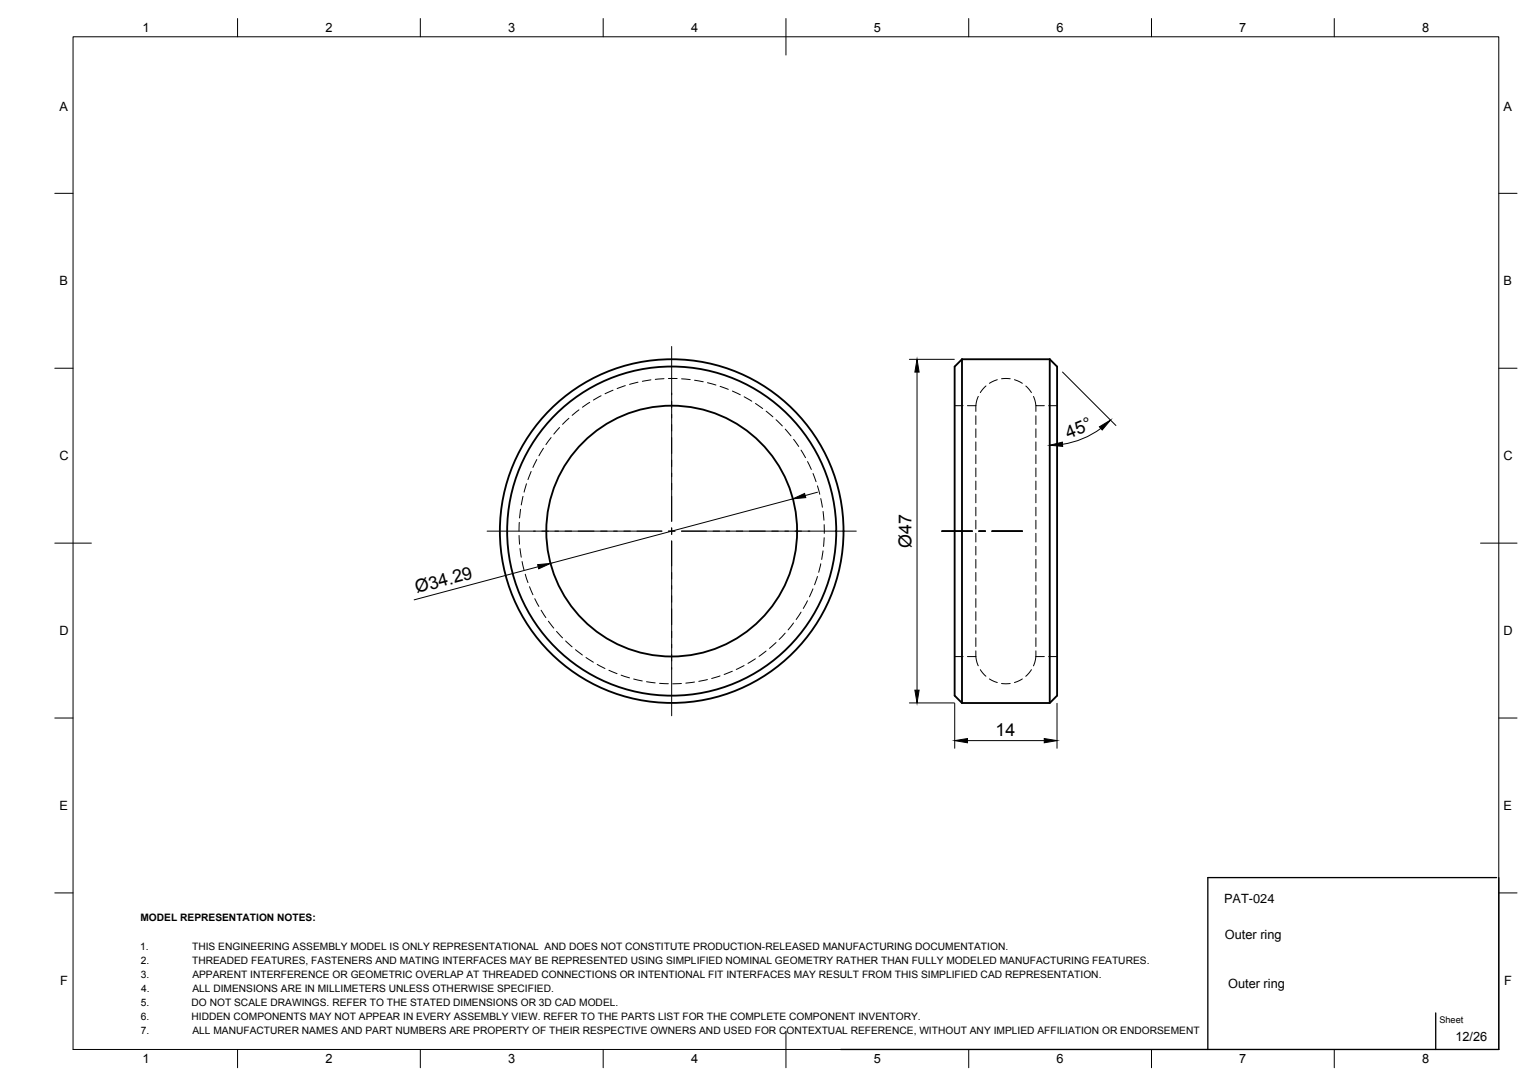
ISO-10303-21;
HEADER;
/* Generated by software containing ST-Developer
 * from STEP Tools, Inc. (www.steptools.com) 
 */

FILE_DESCRIPTION(
/* description */ ('Compact handwheel screw vise'),
/* implementation_level */ '2;1');

FILE_NAME(
/* name */ 'Outer ring.step',
/* time_stamp */ '2026-10-29T16:08:22-07:00',
/* author */ (''),
/* organization */ (''),
/* preprocessor_version */ 'ST-DEVELOPER v20.2',
/* originating_system */ 'Autodesk Translation Framework v15.17.0.0',
/* authorisation */ '');

FILE_SCHEMA (('AUTOMOTIVE_DESIGN { 1 0 10303 214 3 1 1 }'));
ENDSEC;

DATA;
#10=MECHANICAL_DESIGN_GEOMETRIC_PRESENTATION_REPRESENTATION('',(#652),#25074);
#558=TOROIDAL_SURFACE('',#8594,1.675,0.412776);
#564=CONICAL_SURFACE('',#8605,2.3,0.785398163397449);
#565=CONICAL_SURFACE('',#8609,2.3,0.785398163397449);
#596=SHAPE_REPRESENTATION_RELATIONSHIP('SRR','None',#25205,#624);
#624=ADVANCED_BREP_SHAPE_REPRESENTATION('',(#687),#25052);
#652=STYLED_ITEM('',(#25439),#687);
#687=MANIFOLD_SOLID_BREP('Body1',#8061);
#762=FACE_BOUND('',#1636,.T.);
#763=FACE_BOUND('',#1641,.T.);
#881=PLANE('',#8602);
#882=PLANE('',#8611);
#1113=FACE_OUTER_BOUND('',#1633,.T.);
#1114=FACE_OUTER_BOUND('',#1634,.T.);
#1115=FACE_OUTER_BOUND('',#1635,.T.);
#1116=FACE_OUTER_BOUND('',#1637,.T.);
#1117=FACE_OUTER_BOUND('',#1638,.T.);
#1118=FACE_OUTER_BOUND('',#1639,.T.);
#1119=FACE_OUTER_BOUND('',#1640,.T.);
#1120=FACE_OUTER_BOUND('',#1642,.T.);
#1633=EDGE_LOOP('',(#5563,#5564,#5565,#5566,#5567,#5568));
#1634=EDGE_LOOP('',(#5569,#5570,#5571,#5572,#5573));
#1635=EDGE_LOOP('',(#5574));
#1636=EDGE_LOOP('',(#5575));
#1637=EDGE_LOOP('',(#5576,#5577,#5578,#5579));
#1638=EDGE_LOOP('',(#5580,#5581,#5582,#5583));
#1639=EDGE_LOOP('',(#5584,#5585,#5586,#5587));
#1640=EDGE_LOOP('',(#5588));
#1641=EDGE_LOOP('',(#5589));
#1642=EDGE_LOOP('',(#5590,#5591,#5592,#5593,#5594));
#2184=LINE('',#11779,#2692);
#2185=LINE('',#11788,#2693);
#2186=LINE('',#11792,#2694);
#2187=LINE('',#11796,#2695);
#2188=LINE('',#11799,#2696);
#2692=VECTOR('',#9728,1.71469);
#2693=VECTOR('',#9739,2.3);
#2694=VECTOR('',#9744,2.35);
#2695=VECTOR('',#9749,2.3);
#2696=VECTOR('',#9754,1.71469);
#3158=CIRCLE('',#8595,1.71469);
#3159=CIRCLE('',#8596,1.71469);
#3160=CIRCLE('',#8597,0.412776);
#3161=CIRCLE('',#8598,1.71469);
#3162=CIRCLE('',#8599,1.71469);
#3163=CIRCLE('',#8601,1.71469);
#3164=CIRCLE('',#8603,2.25);
#3165=CIRCLE('',#8604,1.71469);
#3166=CIRCLE('',#8606,2.35);
#3167=CIRCLE('',#8608,2.35);
#3168=CIRCLE('',#8610,2.25);
#3466=VERTEX_POINT('',#11767);
#3467=VERTEX_POINT('',#11768);
#3468=VERTEX_POINT('',#11771);
#3469=VERTEX_POINT('',#11773);
#3470=VERTEX_POINT('',#11777);
#3471=VERTEX_POINT('',#11781);
#3472=VERTEX_POINT('',#11783);
#3473=VERTEX_POINT('',#11786);
#3474=VERTEX_POINT('',#11790);
#3475=VERTEX_POINT('',#11794);
#4268=EDGE_CURVE('',#3466,#3467,#3158,.T.);
#4269=EDGE_CURVE('',#3467,#3466,#3159,.T.);
#4270=EDGE_CURVE('',#3467,#3468,#3160,.T.);
#4271=EDGE_CURVE('',#3469,#3468,#3161,.T.);
#4272=EDGE_CURVE('',#3468,#3469,#3162,.T.);
#4273=EDGE_CURVE('',#3470,#3470,#3163,.T.);
#4274=EDGE_CURVE('',#3470,#3469,#2184,.T.);
#4275=EDGE_CURVE('',#3471,#3471,#3164,.T.);
#4276=EDGE_CURVE('',#3472,#3472,#3165,.T.);
#4277=EDGE_CURVE('',#3473,#3473,#3166,.T.);
#4278=EDGE_CURVE('',#3473,#3471,#2185,.T.);
#4279=EDGE_CURVE('',#3474,#3474,#3167,.T.);
#4280=EDGE_CURVE('',#3474,#3473,#2186,.T.);
#4281=EDGE_CURVE('',#3475,#3475,#3168,.T.);
#4282=EDGE_CURVE('',#3475,#3474,#2187,.T.);
#4283=EDGE_CURVE('',#3466,#3472,#2188,.T.);
#5563=ORIENTED_EDGE('',*,*,#4268,.F.);
#5564=ORIENTED_EDGE('',*,*,#4269,.F.);
#5565=ORIENTED_EDGE('',*,*,#4270,.T.);
#5566=ORIENTED_EDGE('',*,*,#4271,.F.);
#5567=ORIENTED_EDGE('',*,*,#4272,.F.);
#5568=ORIENTED_EDGE('',*,*,#4270,.F.);
#5569=ORIENTED_EDGE('',*,*,#4273,.T.);
#5570=ORIENTED_EDGE('',*,*,#4274,.T.);
#5571=ORIENTED_EDGE('',*,*,#4271,.T.);
#5572=ORIENTED_EDGE('',*,*,#4272,.T.);
#5573=ORIENTED_EDGE('',*,*,#4274,.F.);
#5574=ORIENTED_EDGE('',*,*,#4275,.F.);
#5575=ORIENTED_EDGE('',*,*,#4276,.T.);
#5576=ORIENTED_EDGE('',*,*,#4277,.F.);
#5577=ORIENTED_EDGE('',*,*,#4278,.T.);
#5578=ORIENTED_EDGE('',*,*,#4275,.T.);
#5579=ORIENTED_EDGE('',*,*,#4278,.F.);
#5580=ORIENTED_EDGE('',*,*,#4279,.F.);
#5581=ORIENTED_EDGE('',*,*,#4280,.T.);
#5582=ORIENTED_EDGE('',*,*,#4277,.T.);
#5583=ORIENTED_EDGE('',*,*,#4280,.F.);
#5584=ORIENTED_EDGE('',*,*,#4281,.F.);
#5585=ORIENTED_EDGE('',*,*,#4282,.T.);
#5586=ORIENTED_EDGE('',*,*,#4279,.T.);
#5587=ORIENTED_EDGE('',*,*,#4282,.F.);
#5588=ORIENTED_EDGE('',*,*,#4281,.T.);
#5589=ORIENTED_EDGE('',*,*,#4273,.F.);
#5590=ORIENTED_EDGE('',*,*,#4268,.T.);
#5591=ORIENTED_EDGE('',*,*,#4269,.T.);
#5592=ORIENTED_EDGE('',*,*,#4283,.T.);
#5593=ORIENTED_EDGE('',*,*,#4276,.F.);
#5594=ORIENTED_EDGE('',*,*,#4283,.F.);
#7381=CYLINDRICAL_SURFACE('',#8600,1.71469);
#7382=CYLINDRICAL_SURFACE('',#8607,2.35);
#7383=CYLINDRICAL_SURFACE('',#8612,1.71469);
#7683=ADVANCED_FACE('',(#1113),#558,.F.);
#7684=ADVANCED_FACE('',(#1114),#7381,.F.);
#7685=ADVANCED_FACE('',(#1115,#762),#881,.T.);
#7686=ADVANCED_FACE('',(#1116),#564,.T.);
#7687=ADVANCED_FACE('',(#1117),#7382,.T.);
#7688=ADVANCED_FACE('',(#1118),#565,.T.);
#7689=ADVANCED_FACE('',(#1119,#763),#882,.T.);
#7690=ADVANCED_FACE('',(#1120),#7383,.F.);
#8061=CLOSED_SHELL('',(#7683,#7684,#7685,#7686,#7687,#7688,#7689,#7690));
#8593=AXIS2_PLACEMENT_3D('',#11765,#9710,#9711);
#8594=AXIS2_PLACEMENT_3D('',#11766,#9712,#9713);
#8595=AXIS2_PLACEMENT_3D('',#11769,#9714,#9715);
#8596=AXIS2_PLACEMENT_3D('',#11770,#9716,#9717);
#8597=AXIS2_PLACEMENT_3D('',#11772,#9718,#9719);
#8598=AXIS2_PLACEMENT_3D('',#11774,#9720,#9721);
#8599=AXIS2_PLACEMENT_3D('',#11775,#9722,#9723);
#8600=AXIS2_PLACEMENT_3D('',#11776,#9724,#9725);
#8601=AXIS2_PLACEMENT_3D('',#11778,#9726,#9727);
#8602=AXIS2_PLACEMENT_3D('',#11780,#9729,#9730);
#8603=AXIS2_PLACEMENT_3D('',#11782,#9731,#9732);
#8604=AXIS2_PLACEMENT_3D('',#11784,#9733,#9734);
#8605=AXIS2_PLACEMENT_3D('',#11785,#9735,#9736);
#8606=AXIS2_PLACEMENT_3D('',#11787,#9737,#9738);
#8607=AXIS2_PLACEMENT_3D('',#11789,#9740,#9741);
#8608=AXIS2_PLACEMENT_3D('',#11791,#9742,#9743);
#8609=AXIS2_PLACEMENT_3D('',#11793,#9745,#9746);
#8610=AXIS2_PLACEMENT_3D('',#11795,#9747,#9748);
#8611=AXIS2_PLACEMENT_3D('',#11797,#9750,#9751);
#8612=AXIS2_PLACEMENT_3D('',#11798,#9752,#9753);
#9710=DIRECTION('axis',(0.,0.,1.));
#9711=DIRECTION('refdir',(1.,0.,0.));
#9712=DIRECTION('center_axis',(0.,-1.,0.));
#9713=DIRECTION('ref_axis',(0.,0.,-1.));
#9714=DIRECTION('center_axis',(0.,-1.,0.));
#9715=DIRECTION('ref_axis',(1.,0.,0.));
#9716=DIRECTION('center_axis',(0.,-1.,0.));
#9717=DIRECTION('ref_axis',(1.,0.,0.));
#9718=DIRECTION('center_axis',(1.,0.,1.22464679914735E-16));
#9719=DIRECTION('ref_axis',(-1.22464679914735E-16,0.,1.));
#9720=DIRECTION('center_axis',(0.,1.,0.));
#9721=DIRECTION('ref_axis',(1.,0.,0.));
#9722=DIRECTION('center_axis',(0.,1.,0.));
#9723=DIRECTION('ref_axis',(1.,0.,0.));
#9724=DIRECTION('center_axis',(0.,-1.,0.));
#9725=DIRECTION('ref_axis',(1.,0.,0.));
#9726=DIRECTION('center_axis',(0.,-1.,0.));
#9727=DIRECTION('ref_axis',(1.,0.,0.));
#9728=DIRECTION('',(0.,1.,0.));
#9729=DIRECTION('center_axis',(0.,1.,0.));
#9730=DIRECTION('ref_axis',(0.,0.,1.));
#9731=DIRECTION('center_axis',(0.,-1.,0.));
#9732=DIRECTION('ref_axis',(1.,0.,0.));
#9733=DIRECTION('center_axis',(0.,-1.,0.));
#9734=DIRECTION('ref_axis',(1.,0.,0.));
#9735=DIRECTION('center_axis',(0.,-1.,0.));
#9736=DIRECTION('ref_axis',(1.,0.,0.));
#9737=DIRECTION('center_axis',(0.,-1.,0.));
#9738=DIRECTION('ref_axis',(1.,0.,0.));
#9739=DIRECTION('',(0.707106781186548,0.707106781186547,8.65956056235494E-17));
#9740=DIRECTION('center_axis',(0.,-1.,0.));
#9741=DIRECTION('ref_axis',(1.,0.,0.));
#9742=DIRECTION('center_axis',(0.,-1.,0.));
#9743=DIRECTION('ref_axis',(1.,0.,0.));
#9744=DIRECTION('',(0.,1.,0.));
#9745=DIRECTION('center_axis',(0.,1.,0.));
#9746=DIRECTION('ref_axis',(1.,0.,0.));
#9747=DIRECTION('center_axis',(0.,-1.,0.));
#9748=DIRECTION('ref_axis',(1.,0.,0.));
#9749=DIRECTION('',(-0.707106781186548,0.707106781186547,-8.65956056235494E-17));
#9750=DIRECTION('center_axis',(0.,-1.,0.));
#9751=DIRECTION('ref_axis',(0.,0.,-1.));
#9752=DIRECTION('center_axis',(0.,-1.,0.));
#9753=DIRECTION('ref_axis',(1.,0.,0.));
#9754=DIRECTION('',(0.,1.,0.));
#11765=CARTESIAN_POINT('',(0.,0.,0.));
#11766=CARTESIAN_POINT('Origin',(0.,0.,0.));
#11767=CARTESIAN_POINT('',(-1.71469,0.410863395882378,-2.09988962002998E-16));
#11768=CARTESIAN_POINT('',(-2.09988962002998E-16,0.410863395882378,1.71469));
#11769=CARTESIAN_POINT('Origin',(0.,0.410863395882378,0.));
#11770=CARTESIAN_POINT('Origin',(0.,0.410863395882378,0.));
#11771=CARTESIAN_POINT('',(-2.09988962002998E-16,-0.410863395882378,1.71469));
#11772=CARTESIAN_POINT('Origin',(-2.05128338857182E-16,0.,1.675));
#11773=CARTESIAN_POINT('',(-1.71469,-0.410863395882378,2.09988962002998E-16));
#11774=CARTESIAN_POINT('Origin',(0.,-0.410863395882378,0.));
#11775=CARTESIAN_POINT('Origin',(0.,-0.410863395882378,0.));
#11776=CARTESIAN_POINT('Origin',(0.,0.,0.));
#11777=CARTESIAN_POINT('',(-1.71469,-0.7,-2.09988962002998E-16));
#11778=CARTESIAN_POINT('Origin',(0.,-0.7,0.));
#11779=CARTESIAN_POINT('',(-1.71469,0.,-2.09988962002998E-16));
#11780=CARTESIAN_POINT('Origin',(2.25,0.7,0.));
#11781=CARTESIAN_POINT('',(-2.25,0.7,-2.75545529808154E-16));
#11782=CARTESIAN_POINT('Origin',(0.,0.7,0.));
#11783=CARTESIAN_POINT('',(-1.71469,0.7,-2.09988962002998E-16));
#11784=CARTESIAN_POINT('Origin',(0.,0.7,0.));
#11785=CARTESIAN_POINT('Origin',(0.,0.65,0.));
#11786=CARTESIAN_POINT('',(-2.35,0.6,-2.87791997799628E-16));
#11787=CARTESIAN_POINT('Origin',(0.,0.6,0.));
#11788=CARTESIAN_POINT('',(-2.3,0.65,-2.81668763803891E-16));
#11789=CARTESIAN_POINT('Origin',(0.,0.,0.));
#11790=CARTESIAN_POINT('',(-2.35,-0.6,-2.87791997799628E-16));
#11791=CARTESIAN_POINT('Origin',(0.,-0.6,0.));
#11792=CARTESIAN_POINT('',(-2.35,0.,-2.87791997799628E-16));
#11793=CARTESIAN_POINT('Origin',(0.,-0.65,0.));
#11794=CARTESIAN_POINT('',(-2.25,-0.7,-2.75545529808154E-16));
#11795=CARTESIAN_POINT('Origin',(0.,-0.7,0.));
#11796=CARTESIAN_POINT('',(-2.3,-0.65,-2.81668763803891E-16));
#11797=CARTESIAN_POINT('Origin',(1.71469,-0.7,0.));
#11798=CARTESIAN_POINT('Origin',(0.,0.,0.));
#11799=CARTESIAN_POINT('',(-1.71469,0.,-2.09988962002998E-16));
#25018=UNCERTAINTY_MEASURE_WITH_UNIT(LENGTH_MEASURE(0.001),#25075,
'DISTANCE_ACCURACY_VALUE',
'Maximum model space distance between geometric entities at asserted c
onnectivities');
#25040=UNCERTAINTY_MEASURE_WITH_UNIT(LENGTH_MEASURE(0.001),#25075,
'DISTANCE_ACCURACY_VALUE',
'Maximum model space distance between geometric entities at asserted c
onnectivities');
#25052=(
GEOMETRIC_REPRESENTATION_CONTEXT(3)
GLOBAL_UNCERTAINTY_ASSIGNED_CONTEXT((#25018))
GLOBAL_UNIT_ASSIGNED_CONTEXT((#25075,#25077,#25078))
REPRESENTATION_CONTEXT('','3D')
);
#25074=(
GEOMETRIC_REPRESENTATION_CONTEXT(3)
GLOBAL_UNCERTAINTY_ASSIGNED_CONTEXT((#25040))
GLOBAL_UNIT_ASSIGNED_CONTEXT((#25075,#25077,#25078))
REPRESENTATION_CONTEXT('','3D')
);
#25075=(
LENGTH_UNIT()
NAMED_UNIT(*)
SI_UNIT(.CENTI.,.METRE.)
);
#25077=(
NAMED_UNIT(*)
PLANE_ANGLE_UNIT()
SI_UNIT($,.RADIAN.)
);
#25078=(
NAMED_UNIT(*)
SI_UNIT($,.STERADIAN.)
SOLID_ANGLE_UNIT()
);
#25090=SHAPE_DEFINITION_REPRESENTATION(#25123,#25205);
#25123=PRODUCT_DEFINITION_SHAPE('',$,#25239);
#25205=SHAPE_REPRESENTATION('',(#8593),#25052);
#25227=PRODUCT_DEFINITION_CONTEXT('part definition',#25328,'design');
#25239=PRODUCT_DEFINITION('Outer ring','Outer ring',#25272,#25227);
#25272=PRODUCT_DEFINITION_FORMATION('',$,#25341);
#25328=APPLICATION_CONTEXT(
'Core Data for Automotive Mechanical Design Process');
#25329=PRODUCT_CONTEXT('part definition',#25328,'mechanical');
#25341=PRODUCT('Outer ring','Outer ring','Outer ring',(#25329));
#25433=COLOUR_RGB('Grey',0.48,0.52,0.57);
#25434=FILL_AREA_STYLE_COLOUR('',#25433);
#25435=FILL_AREA_STYLE('',(#25434));
#25436=SURFACE_STYLE_FILL_AREA(#25435);
#25437=SURFACE_SIDE_STYLE('',(#25436));
#25438=SURFACE_STYLE_USAGE(.BOTH.,#25437);
#25439=PRESENTATION_STYLE_ASSIGNMENT((#25438));
ENDSEC;
END-ISO-10303-21;
